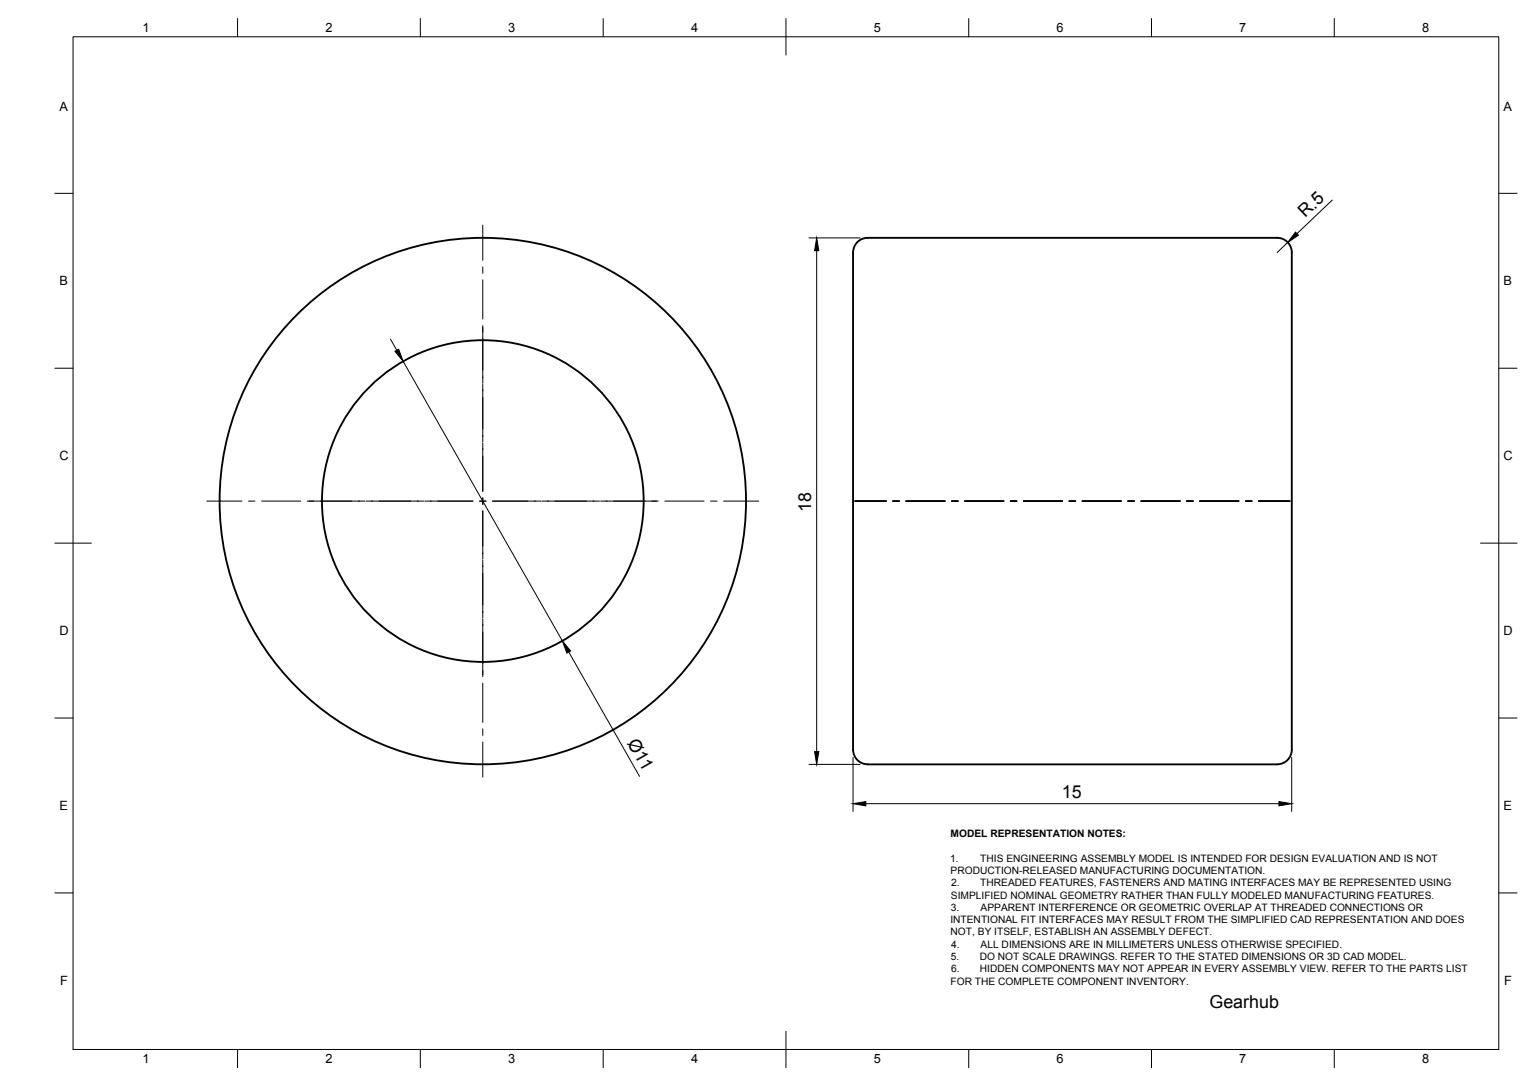
ISO-10303-21;
HEADER;
/* Generated by software containing ST-Developer
 * from STEP Tools, Inc. (www.steptools.com) 
 */

FILE_DESCRIPTION(
/* description */ ('STEP AP242 Edition 2'),
/* implementation_level */ '2;1');

FILE_NAME(
/* name */ 'Gearhub.step',
/* time_stamp */ '2026-10-06T10:11:12-07:00',
/* author */ (''),
/* organization */ (''),
/* preprocessor_version */ 'ST-DEVELOPER v20.2',
/* originating_system */ 'Autodesk Translation Framework v15.15.0.0',
/* authorisation */ '');

FILE_SCHEMA (('AUTOMOTIVE_DESIGN { 1 0 10303 214 3 1 1 }'));
ENDSEC;

DATA;
#10=MECHANICAL_DESIGN_GEOMETRIC_PRESENTATION_REPRESENTATION('',(#1795),#54580);
#258=TOROIDAL_SURFACE('',#19075,0.0085,0.0005);
#259=TOROIDAL_SURFACE('',#19077,0.0085,0.0005);
#1751=SHAPE_REPRESENTATION_RELATIONSHIP('SRR','None',#54638,#1765);
#1765=ADVANCED_BREP_SHAPE_REPRESENTATION('',(#1809),#54574);
#1795=STYLED_ITEM('',(#54709),#1809);
#1809=MANIFOLD_SOLID_BREP('Body1',#17674);
#2260=LINE('',#48568,#2853);
#2261=LINE('',#48576,#2854);
#2853=VECTOR('',#22516,0.009);
#2854=VECTOR('',#22527,0.0055);
#3398=CYLINDRICAL_SURFACE('',#19067,0.009);
#3399=CYLINDRICAL_SURFACE('',#19074,0.0055);
#3511=FACE_BOUND('',#5336,.T.);
#3512=FACE_BOUND('',#5339,.T.);
#4295=FACE_OUTER_BOUND('',#5335,.T.);
#4296=FACE_OUTER_BOUND('',#5337,.T.);
#4297=FACE_OUTER_BOUND('',#5338,.T.);
#4298=FACE_OUTER_BOUND('',#5340,.T.);
#4299=FACE_OUTER_BOUND('',#5341,.T.);
#4300=FACE_OUTER_BOUND('',#5342,.T.);
#5335=EDGE_LOOP('',(#15303));
#5336=EDGE_LOOP('',(#15304));
#5337=EDGE_LOOP('',(#15305,#15306,#15307,#15308,#15309));
#5338=EDGE_LOOP('',(#15310));
#5339=EDGE_LOOP('',(#15311));
#5340=EDGE_LOOP('',(#15312,#15313,#15314,#15315));
#5341=EDGE_LOOP('',(#15316,#15317,#15318,#15319));
#5342=EDGE_LOOP('',(#15320,#15321,#15322,#15323,#15324));
#6233=CIRCLE('',#19065,0.0085);
#6234=CIRCLE('',#19066,0.0055);
#6235=CIRCLE('',#19068,0.009);
#6236=CIRCLE('',#19069,0.009);
#6237=CIRCLE('',#19070,0.009);
#6238=CIRCLE('',#19072,0.0085);
#6239=CIRCLE('',#19073,0.0055);
#6240=CIRCLE('',#19076,0.0005);
#6241=CIRCLE('',#19078,0.0005);
#7934=VERTEX_POINT('',#48558);
#7935=VERTEX_POINT('',#48560);
#7936=VERTEX_POINT('',#48563);
#7937=VERTEX_POINT('',#48564);
#7938=VERTEX_POINT('',#48567);
#7939=VERTEX_POINT('',#48571);
#7940=VERTEX_POINT('',#48573);
#10443=EDGE_CURVE('',#7934,#7934,#6233,.F.);
#10444=EDGE_CURVE('',#7935,#7935,#6234,.T.);
#10445=EDGE_CURVE('',#7936,#7937,#6235,.T.);
#10446=EDGE_CURVE('',#7937,#7936,#6236,.T.);
#10447=EDGE_CURVE('',#7936,#7938,#2260,.T.);
#10448=EDGE_CURVE('',#7938,#7938,#6237,.T.);
#10449=EDGE_CURVE('',#7939,#7939,#6238,.F.);
#10450=EDGE_CURVE('',#7940,#7940,#6239,.T.);
#10451=EDGE_CURVE('',#7940,#7935,#2261,.T.);
#10452=EDGE_CURVE('',#7938,#7939,#6240,.T.);
#10453=EDGE_CURVE('',#7937,#7934,#6241,.T.);
#15303=ORIENTED_EDGE('',*,*,#10443,.T.);
#15304=ORIENTED_EDGE('',*,*,#10444,.T.);
#15305=ORIENTED_EDGE('',*,*,#10445,.T.);
#15306=ORIENTED_EDGE('',*,*,#10446,.T.);
#15307=ORIENTED_EDGE('',*,*,#10447,.T.);
#15308=ORIENTED_EDGE('',*,*,#10448,.T.);
#15309=ORIENTED_EDGE('',*,*,#10447,.F.);
#15310=ORIENTED_EDGE('',*,*,#10449,.T.);
#15311=ORIENTED_EDGE('',*,*,#10450,.T.);
#15312=ORIENTED_EDGE('',*,*,#10450,.F.);
#15313=ORIENTED_EDGE('',*,*,#10451,.T.);
#15314=ORIENTED_EDGE('',*,*,#10444,.F.);
#15315=ORIENTED_EDGE('',*,*,#10451,.F.);
#15316=ORIENTED_EDGE('',*,*,#10448,.F.);
#15317=ORIENTED_EDGE('',*,*,#10452,.T.);
#15318=ORIENTED_EDGE('',*,*,#10449,.F.);
#15319=ORIENTED_EDGE('',*,*,#10452,.F.);
#15320=ORIENTED_EDGE('',*,*,#10445,.F.);
#15321=ORIENTED_EDGE('',*,*,#10446,.F.);
#15322=ORIENTED_EDGE('',*,*,#10453,.T.);
#15323=ORIENTED_EDGE('',*,*,#10443,.F.);
#15324=ORIENTED_EDGE('',*,*,#10453,.F.);
#16612=PLANE('',#19064);
#16613=PLANE('',#19071);
#17411=ADVANCED_FACE('',(#4295,#3511),#16612,.F.);
#17412=ADVANCED_FACE('',(#4296),#3398,.T.);
#17413=ADVANCED_FACE('',(#4297,#3512),#16613,.F.);
#17414=ADVANCED_FACE('',(#4298),#3399,.F.);
#17415=ADVANCED_FACE('',(#4299),#258,.T.);
#17416=ADVANCED_FACE('',(#4300),#259,.T.);
#17674=CLOSED_SHELL('',(#17411,#17412,#17413,#17414,#17415,#17416));
#19063=AXIS2_PLACEMENT_3D('',#48556,#22502,#22503);
#19064=AXIS2_PLACEMENT_3D('',#48557,#22504,#22505);
#19065=AXIS2_PLACEMENT_3D('',#48559,#22506,#22507);
#19066=AXIS2_PLACEMENT_3D('',#48561,#22508,#22509);
#19067=AXIS2_PLACEMENT_3D('',#48562,#22510,#22511);
#19068=AXIS2_PLACEMENT_3D('',#48565,#22512,#22513);
#19069=AXIS2_PLACEMENT_3D('',#48566,#22514,#22515);
#19070=AXIS2_PLACEMENT_3D('',#48569,#22517,#22518);
#19071=AXIS2_PLACEMENT_3D('',#48570,#22519,#22520);
#19072=AXIS2_PLACEMENT_3D('',#48572,#22521,#22522);
#19073=AXIS2_PLACEMENT_3D('',#48574,#22523,#22524);
#19074=AXIS2_PLACEMENT_3D('',#48575,#22525,#22526);
#19075=AXIS2_PLACEMENT_3D('',#48577,#22528,#22529);
#19076=AXIS2_PLACEMENT_3D('',#48578,#22530,#22531);
#19077=AXIS2_PLACEMENT_3D('',#48579,#22532,#22533);
#19078=AXIS2_PLACEMENT_3D('',#48580,#22534,#22535);
#22502=DIRECTION('axis',(0.,0.,1.));
#22503=DIRECTION('refdir',(1.,0.,0.));
#22504=DIRECTION('center_axis',(1.33376816360845E-16,-1.,0.));
#22505=DIRECTION('ref_axis',(1.,1.33376816360845E-16,0.));
#22506=DIRECTION('center_axis',(1.33376816360845E-16,-1.,0.));
#22507=DIRECTION('ref_axis',(1.,1.33376816360845E-16,0.));
#22508=DIRECTION('center_axis',(1.33376816360845E-16,-1.,0.));
#22509=DIRECTION('ref_axis',(1.,1.33376816360845E-16,0.));
#22510=DIRECTION('center_axis',(-1.33376816360845E-16,1.,0.));
#22511=DIRECTION('ref_axis',(-1.,-1.33376816360845E-16,0.));
#22512=DIRECTION('center_axis',(1.33376816360845E-16,-1.,0.));
#22513=DIRECTION('ref_axis',(1.,1.33376816360845E-16,0.));
#22514=DIRECTION('center_axis',(1.33376816360845E-16,-1.,0.));
#22515=DIRECTION('ref_axis',(1.,1.33376816360845E-16,0.));
#22516=DIRECTION('',(1.33376816360845E-16,-1.,0.));
#22517=DIRECTION('center_axis',(-1.33376816360845E-16,1.,0.));
#22518=DIRECTION('ref_axis',(-1.,-1.33376816360845E-16,0.));
#22519=DIRECTION('center_axis',(-1.33376816360845E-16,1.,0.));
#22520=DIRECTION('ref_axis',(-1.,-1.33376816360845E-16,0.));
#22521=DIRECTION('center_axis',(-1.33376816360845E-16,1.,0.));
#22522=DIRECTION('ref_axis',(-1.,-1.33376816360845E-16,0.));
#22523=DIRECTION('center_axis',(-1.33376816360845E-16,1.,0.));
#22524=DIRECTION('ref_axis',(-1.,-1.33376816360845E-16,0.));
#22525=DIRECTION('center_axis',(-1.33376816360845E-16,1.,0.));
#22526=DIRECTION('ref_axis',(-1.,-1.33376816360845E-16,0.));
#22527=DIRECTION('',(-1.33376816360845E-16,1.,0.));
#22528=DIRECTION('center_axis',(-1.33376816360845E-16,1.,0.));
#22529=DIRECTION('ref_axis',(-1.,-1.32513598859339E-16,0.));
#22530=DIRECTION('center_axis',(-1.22464679914735E-16,-1.63339491236773E-32,
-1.));
#22531=DIRECTION('ref_axis',(1.,1.31067995962692E-16,-1.22464679914735E-16));
#22532=DIRECTION('center_axis',(1.33376816360845E-16,-1.,0.));
#22533=DIRECTION('ref_axis',(1.,1.92747052886312E-16,0.));
#22534=DIRECTION('center_axis',(1.22464679914735E-16,1.63339491236773E-32,
-1.));
#22535=DIRECTION('ref_axis',(-1.,-2.46716227694479E-16,-1.22464679914735E-16));
#48556=CARTESIAN_POINT('',(0.,0.,0.));
#48557=CARTESIAN_POINT('Origin',(0.00475,0.014,0.));
#48558=CARTESIAN_POINT('',(-0.0085,0.014,-1.04094977927525E-18));
#48559=CARTESIAN_POINT('Origin',(1.20286593710508E-18,0.014,0.));
#48560=CARTESIAN_POINT('',(0.0055,0.014,0.));
#48561=CARTESIAN_POINT('Origin',(-1.86727542905183E-18,0.014,0.));
#48562=CARTESIAN_POINT('Origin',(0.,0.0230185533732548,0.));
#48563=CARTESIAN_POINT('',(0.009,0.0135,0.));
#48564=CARTESIAN_POINT('',(-0.009,0.0135,-1.10218211923262E-18));
#48565=CARTESIAN_POINT('Origin',(1.2695543452855E-18,0.0135,0.));
#48566=CARTESIAN_POINT('Origin',(1.2695543452855E-18,0.0135,0.));
#48567=CARTESIAN_POINT('',(0.009,-0.000500000000000003,-1.10218211923262E-18));
#48568=CARTESIAN_POINT('',(0.009,0.0230185533732548,-1.10218211923262E-18));
#48569=CARTESIAN_POINT('Origin',(3.13682977433732E-18,-0.0005,0.));
#48570=CARTESIAN_POINT('Origin',(0.009,-0.001,0.));
#48571=CARTESIAN_POINT('',(0.0085,-0.000999999999999999,-1.04094977927525E-18));
#48572=CARTESIAN_POINT('Origin',(3.20351818251775E-18,-0.001,0.));
#48573=CARTESIAN_POINT('',(0.0055,-0.001,-6.73555739531044E-19));
#48574=CARTESIAN_POINT('Origin',(1.33376816360845E-19,-0.001,0.));
#48575=CARTESIAN_POINT('Origin',(2.13402906177352E-18,-0.016,0.));
#48576=CARTESIAN_POINT('',(0.0055,-0.016,-6.73555739531044E-19));
#48577=CARTESIAN_POINT('Origin',(3.13682977433732E-18,-0.0005,0.));
#48578=CARTESIAN_POINT('Origin',(0.0085,-0.000499999999999999,-1.04094977927525E-18));
#48579=CARTESIAN_POINT('Origin',(1.2695543452855E-18,0.0135,0.));
#48580=CARTESIAN_POINT('Origin',(-0.0085,0.0135,-1.04094977927525E-18));
#54558=UNCERTAINTY_MEASURE_WITH_UNIT(LENGTH_MEASURE(1.E-5),#54581,
'DISTANCE_ACCURACY_VALUE',
'Maximum model space distance between geometric entities at asserted c
onnectivities');
#54564=UNCERTAINTY_MEASURE_WITH_UNIT(LENGTH_MEASURE(1.E-5),#54581,
'DISTANCE_ACCURACY_VALUE',
'Maximum model space distance between geometric entities at asserted c
onnectivities');
#54574=(
GEOMETRIC_REPRESENTATION_CONTEXT(3)
GLOBAL_UNCERTAINTY_ASSIGNED_CONTEXT((#54558))
GLOBAL_UNIT_ASSIGNED_CONTEXT((#54581,#54582,#54583))
REPRESENTATION_CONTEXT('','3D')
);
#54580=(
GEOMETRIC_REPRESENTATION_CONTEXT(3)
GLOBAL_UNCERTAINTY_ASSIGNED_CONTEXT((#54564))
GLOBAL_UNIT_ASSIGNED_CONTEXT((#54581,#54582,#54583))
REPRESENTATION_CONTEXT('','3D')
);
#54581=(
LENGTH_UNIT()
NAMED_UNIT(*)
SI_UNIT($,.METRE.)
);
#54582=(
NAMED_UNIT(*)
PLANE_ANGLE_UNIT()
SI_UNIT($,.RADIAN.)
);
#54583=(
NAMED_UNIT(*)
SI_UNIT($,.STERADIAN.)
SOLID_ANGLE_UNIT()
);
#54593=SHAPE_DEFINITION_REPRESENTATION(#54608,#54638);
#54608=PRODUCT_DEFINITION_SHAPE('',$,#54654);
#54638=SHAPE_REPRESENTATION('',(#19063),#54574);
#54644=PRODUCT_DEFINITION_CONTEXT('part definition',#54691,'design');
#54654=PRODUCT_DEFINITION('gearhub','Gearhub',#54669,#54644);
#54669=PRODUCT_DEFINITION_FORMATION('',$,#54702);
#54691=APPLICATION_CONTEXT(
'Core Data for Automotive Mechanical Design Process');
#54692=PRODUCT_CONTEXT('part definition',#54691,'mechanical');
#54702=PRODUCT('gearhub','Gearhub','gearhub',(#54692));
#54709=PRESENTATION_STYLE_ASSIGNMENT((#54719));
#54719=SURFACE_STYLE_USAGE(.BOTH.,#54729);
#54729=SURFACE_SIDE_STYLE('',(#54739));
#54739=SURFACE_STYLE_FILL_AREA(#54749);
#54749=FILL_AREA_STYLE('Opaque(153,153,153)',(#54759));
#54759=FILL_AREA_STYLE_COLOUR('Opaque(153,153,153)',#54769);
#54769=COLOUR_RGB('Opaque(153,153,153)', 0.09019608, 0.27058824, 0.51372549);
ENDSEC;
END-ISO-10303-21;
